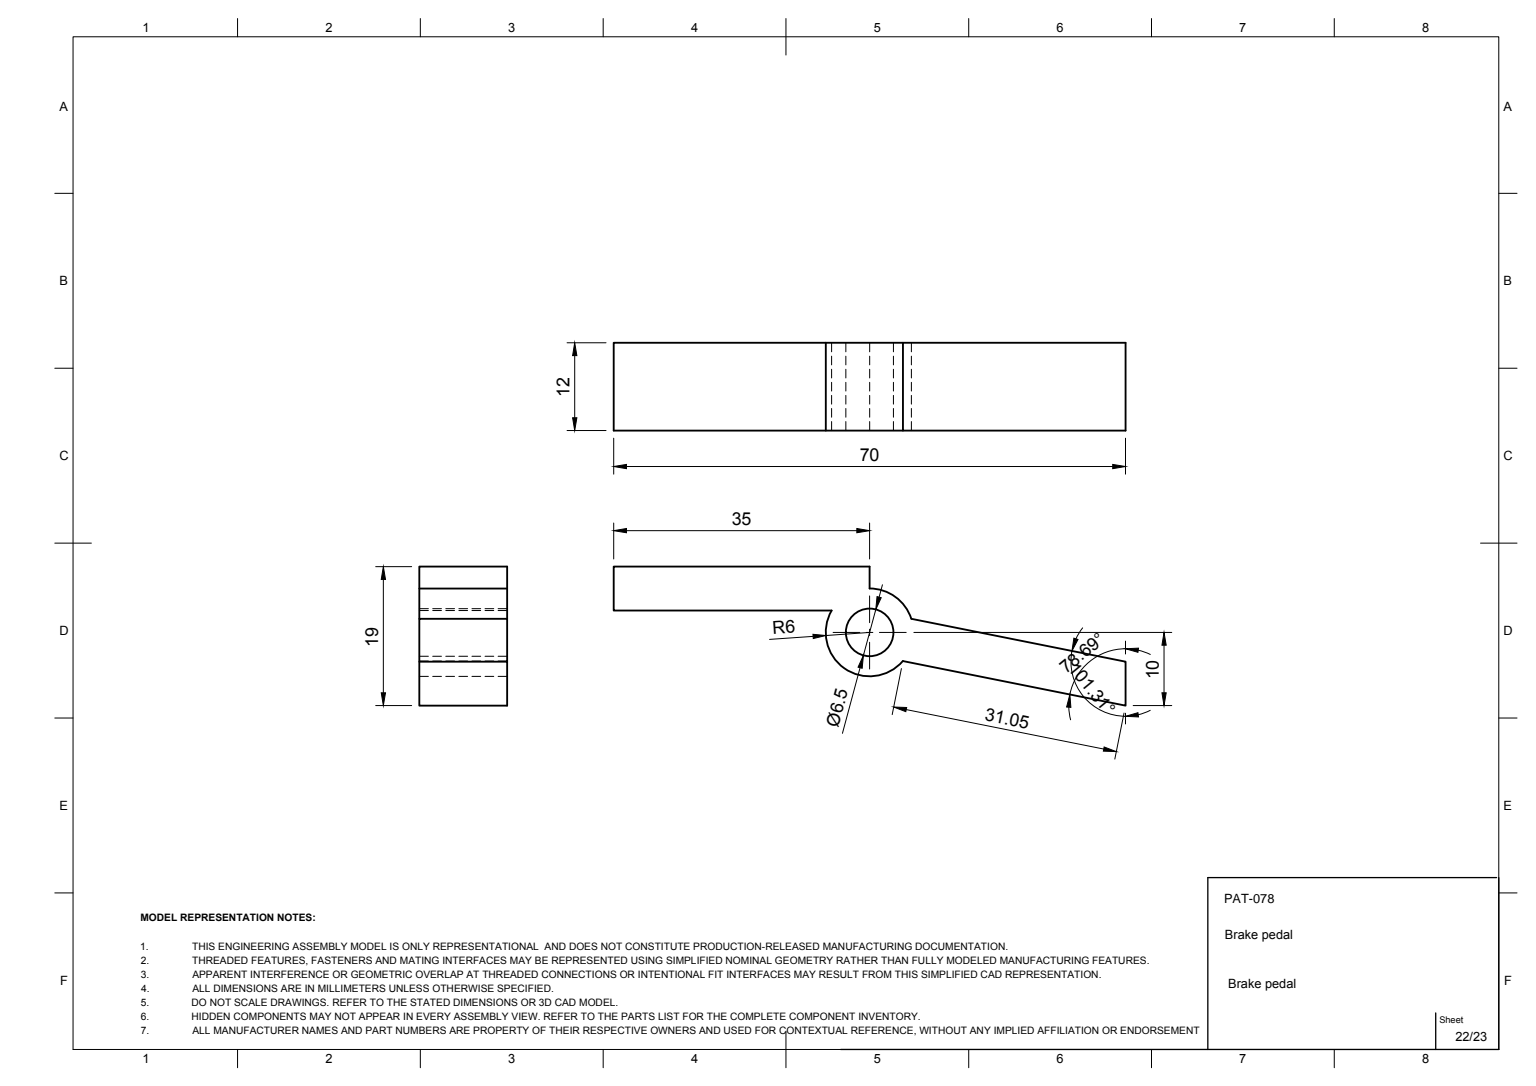
ISO-10303-21;
HEADER;
/* Generated by software containing ST-Developer
 * from STEP Tools, Inc. (www.steptools.com) 
 */

FILE_DESCRIPTION(
/* description */ ('Pedal-braked fixed caster'),
/* implementation_level */ '2;1');

FILE_NAME(
/* name */ 'Brake pedal.step',
/* time_stamp */ '2026-10-28T03:26:52-07:00',
/* author */ (''),
/* organization */ (''),
/* preprocessor_version */ 'ST-DEVELOPER v20.2',
/* originating_system */ 'Autodesk Translation Framework v15.17.0.0',
/* authorisation */ '');

FILE_SCHEMA (('AUTOMOTIVE_DESIGN { 1 0 10303 214 3 1 1 }'));
ENDSEC;

DATA;
#10=MECHANICAL_DESIGN_GEOMETRIC_PRESENTATION_REPRESENTATION('',(#228),#5734);
#187=SHAPE_REPRESENTATION_RELATIONSHIP('SRR','None',#5828,#204);
#204=ADVANCED_BREP_SHAPE_REPRESENTATION('',(#251),#5732);
#228=STYLED_ITEM('',(#5977),#251);
#251=MANIFOLD_SOLID_BREP('Body1',#3010);
#292=CYLINDRICAL_SURFACE('',#3531,0.325);
#293=CYLINDRICAL_SURFACE('',#3540,0.6);
#294=CYLINDRICAL_SURFACE('',#3548,0.6);
#338=FACE_BOUND('',#862,.T.);
#339=FACE_BOUND('',#869,.T.);
#470=CIRCLE('',#3532,0.325);
#471=CIRCLE('',#3533,0.325);
#472=CIRCLE('',#3538,0.6);
#473=CIRCLE('',#3539,0.6);
#474=CIRCLE('',#3541,0.6);
#475=CIRCLE('',#3547,0.6);
#636=FACE_OUTER_BOUND('',#857,.T.);
#637=FACE_OUTER_BOUND('',#858,.T.);
#638=FACE_OUTER_BOUND('',#859,.T.);
#639=FACE_OUTER_BOUND('',#860,.T.);
#640=FACE_OUTER_BOUND('',#861,.T.);
#641=FACE_OUTER_BOUND('',#863,.T.);
#642=FACE_OUTER_BOUND('',#864,.T.);
#643=FACE_OUTER_BOUND('',#865,.T.);
#644=FACE_OUTER_BOUND('',#866,.T.);
#645=FACE_OUTER_BOUND('',#867,.T.);
#646=FACE_OUTER_BOUND('',#868,.T.);
#647=FACE_OUTER_BOUND('',#870,.T.);
#857=EDGE_LOOP('',(#2616,#2617,#2618,#2619));
#858=EDGE_LOOP('',(#2620,#2621,#2622,#2623));
#859=EDGE_LOOP('',(#2624,#2625,#2626,#2627));
#860=EDGE_LOOP('',(#2628,#2629,#2630,#2631));
#861=EDGE_LOOP('',(#2632,#2633,#2634,#2635,#2636,#2637,#2638,#2639,#2640));
#862=EDGE_LOOP('',(#2641));
#863=EDGE_LOOP('',(#2642,#2643,#2644,#2645));
#864=EDGE_LOOP('',(#2646,#2647,#2648,#2649));
#865=EDGE_LOOP('',(#2650,#2651,#2652,#2653));
#866=EDGE_LOOP('',(#2654,#2655,#2656,#2657));
#867=EDGE_LOOP('',(#2658,#2659,#2660,#2661));
#868=EDGE_LOOP('',(#2662,#2663,#2664,#2665,#2666,#2667,#2668,#2669,#2670));
#869=EDGE_LOOP('',(#2671));
#870=EDGE_LOOP('',(#2672,#2673,#2674,#2675));
#1053=LINE('',#5599,#1265);
#1054=LINE('',#5604,#1266);
#1055=LINE('',#5606,#1267);
#1056=LINE('',#5608,#1268);
#1057=LINE('',#5609,#1269);
#1058=LINE('',#5612,#1270);
#1059=LINE('',#5614,#1271);
#1060=LINE('',#5615,#1272);
#1061=LINE('',#5619,#1273);
#1062=LINE('',#5620,#1274);
#1063=LINE('',#5621,#1275);
#1064=LINE('',#5626,#1276);
#1065=LINE('',#5628,#1277);
#1066=LINE('',#5630,#1278);
#1067=LINE('',#5632,#1279);
#1068=LINE('',#5637,#1280);
#1069=LINE('',#5640,#1281);
#1070=LINE('',#5642,#1282);
#1071=LINE('',#5643,#1283);
#1072=LINE('',#5646,#1284);
#1073=LINE('',#5647,#1285);
#1074=LINE('',#5650,#1286);
#1075=LINE('',#5651,#1287);
#1076=LINE('',#5653,#1288);
#1265=VECTOR('',#4403,0.325);
#1266=VECTOR('',#4408,1.);
#1267=VECTOR('',#4409,1.);
#1268=VECTOR('',#4410,1.);
#1269=VECTOR('',#4411,1.);
#1270=VECTOR('',#4414,1.);
#1271=VECTOR('',#4415,1.);
#1272=VECTOR('',#4416,1.);
#1273=VECTOR('',#4419,1.);
#1274=VECTOR('',#4420,1.);
#1275=VECTOR('',#4421,1.);
#1276=VECTOR('',#4426,1.);
#1277=VECTOR('',#4427,1.);
#1278=VECTOR('',#4428,1.);
#1279=VECTOR('',#4429,1.);
#1280=VECTOR('',#4436,1.);
#1281=VECTOR('',#4439,1.);
#1282=VECTOR('',#4440,1.);
#1283=VECTOR('',#4441,1.);
#1284=VECTOR('',#4444,1.);
#1285=VECTOR('',#4445,1.);
#1286=VECTOR('',#4448,1.);
#1287=VECTOR('',#4449,1.);
#1288=VECTOR('',#4452,1.);
#1532=VERTEX_POINT('',#5596);
#1533=VERTEX_POINT('',#5598);
#1534=VERTEX_POINT('',#5602);
#1535=VERTEX_POINT('',#5603);
#1536=VERTEX_POINT('',#5605);
#1537=VERTEX_POINT('',#5607);
#1538=VERTEX_POINT('',#5611);
#1539=VERTEX_POINT('',#5613);
#1540=VERTEX_POINT('',#5617);
#1541=VERTEX_POINT('',#5618);
#1542=VERTEX_POINT('',#5623);
#1543=VERTEX_POINT('',#5625);
#1544=VERTEX_POINT('',#5627);
#1545=VERTEX_POINT('',#5629);
#1546=VERTEX_POINT('',#5631);
#1547=VERTEX_POINT('',#5635);
#1548=VERTEX_POINT('',#5639);
#1549=VERTEX_POINT('',#5641);
#1550=VERTEX_POINT('',#5645);
#1551=VERTEX_POINT('',#5649);
#1898=EDGE_CURVE('',#1532,#1532,#470,.T.);
#1899=EDGE_CURVE('',#1532,#1533,#1053,.T.);
#1900=EDGE_CURVE('',#1533,#1533,#471,.T.);
#1901=EDGE_CURVE('',#1534,#1535,#1054,.T.);
#1902=EDGE_CURVE('',#1536,#1534,#1055,.T.);
#1903=EDGE_CURVE('',#1537,#1536,#1056,.T.);
#1904=EDGE_CURVE('',#1535,#1537,#1057,.T.);
#1905=EDGE_CURVE('',#1537,#1538,#1058,.T.);
#1906=EDGE_CURVE('',#1539,#1536,#1059,.T.);
#1907=EDGE_CURVE('',#1538,#1539,#1060,.T.);
#1908=EDGE_CURVE('',#1540,#1541,#1061,.T.);
#1909=EDGE_CURVE('',#1538,#1540,#1062,.T.);
#1910=EDGE_CURVE('',#1541,#1539,#1063,.T.);
#1911=EDGE_CURVE('',#1542,#1540,#472,.T.);
#1912=EDGE_CURVE('',#1542,#1543,#1064,.T.);
#1913=EDGE_CURVE('',#1543,#1544,#1065,.T.);
#1914=EDGE_CURVE('',#1544,#1545,#1066,.T.);
#1915=EDGE_CURVE('',#1545,#1546,#1067,.T.);
#1916=EDGE_CURVE('',#1535,#1546,#473,.T.);
#1917=EDGE_CURVE('',#1547,#1541,#474,.T.);
#1918=EDGE_CURVE('',#1547,#1542,#1068,.T.);
#1919=EDGE_CURVE('',#1546,#1548,#1069,.T.);
#1920=EDGE_CURVE('',#1545,#1549,#1070,.T.);
#1921=EDGE_CURVE('',#1548,#1549,#1071,.T.);
#1922=EDGE_CURVE('',#1550,#1547,#1072,.T.);
#1923=EDGE_CURVE('',#1543,#1550,#1073,.T.);
#1924=EDGE_CURVE('',#1551,#1550,#1074,.T.);
#1925=EDGE_CURVE('',#1544,#1551,#1075,.T.);
#1926=EDGE_CURVE('',#1549,#1551,#1076,.T.);
#1927=EDGE_CURVE('',#1534,#1548,#475,.T.);
#2616=ORIENTED_EDGE('',*,*,#1898,.F.);
#2617=ORIENTED_EDGE('',*,*,#1899,.T.);
#2618=ORIENTED_EDGE('',*,*,#1900,.F.);
#2619=ORIENTED_EDGE('',*,*,#1899,.F.);
#2620=ORIENTED_EDGE('',*,*,#1901,.F.);
#2621=ORIENTED_EDGE('',*,*,#1902,.F.);
#2622=ORIENTED_EDGE('',*,*,#1903,.F.);
#2623=ORIENTED_EDGE('',*,*,#1904,.F.);
#2624=ORIENTED_EDGE('',*,*,#1905,.F.);
#2625=ORIENTED_EDGE('',*,*,#1903,.T.);
#2626=ORIENTED_EDGE('',*,*,#1906,.F.);
#2627=ORIENTED_EDGE('',*,*,#1907,.F.);
#2628=ORIENTED_EDGE('',*,*,#1908,.F.);
#2629=ORIENTED_EDGE('',*,*,#1909,.F.);
#2630=ORIENTED_EDGE('',*,*,#1907,.T.);
#2631=ORIENTED_EDGE('',*,*,#1910,.F.);
#2632=ORIENTED_EDGE('',*,*,#1911,.F.);
#2633=ORIENTED_EDGE('',*,*,#1912,.T.);
#2634=ORIENTED_EDGE('',*,*,#1913,.T.);
#2635=ORIENTED_EDGE('',*,*,#1914,.T.);
#2636=ORIENTED_EDGE('',*,*,#1915,.T.);
#2637=ORIENTED_EDGE('',*,*,#1916,.F.);
#2638=ORIENTED_EDGE('',*,*,#1904,.T.);
#2639=ORIENTED_EDGE('',*,*,#1905,.T.);
#2640=ORIENTED_EDGE('',*,*,#1909,.T.);
#2641=ORIENTED_EDGE('',*,*,#1898,.T.);
#2642=ORIENTED_EDGE('',*,*,#1908,.T.);
#2643=ORIENTED_EDGE('',*,*,#1917,.F.);
#2644=ORIENTED_EDGE('',*,*,#1918,.T.);
#2645=ORIENTED_EDGE('',*,*,#1911,.T.);
#2646=ORIENTED_EDGE('',*,*,#1919,.F.);
#2647=ORIENTED_EDGE('',*,*,#1915,.F.);
#2648=ORIENTED_EDGE('',*,*,#1920,.T.);
#2649=ORIENTED_EDGE('',*,*,#1921,.F.);
#2650=ORIENTED_EDGE('',*,*,#1918,.F.);
#2651=ORIENTED_EDGE('',*,*,#1922,.F.);
#2652=ORIENTED_EDGE('',*,*,#1923,.F.);
#2653=ORIENTED_EDGE('',*,*,#1912,.F.);
#2654=ORIENTED_EDGE('',*,*,#1913,.F.);
#2655=ORIENTED_EDGE('',*,*,#1923,.T.);
#2656=ORIENTED_EDGE('',*,*,#1924,.F.);
#2657=ORIENTED_EDGE('',*,*,#1925,.F.);
#2658=ORIENTED_EDGE('',*,*,#1914,.F.);
#2659=ORIENTED_EDGE('',*,*,#1925,.T.);
#2660=ORIENTED_EDGE('',*,*,#1926,.F.);
#2661=ORIENTED_EDGE('',*,*,#1920,.F.);
#2662=ORIENTED_EDGE('',*,*,#1927,.T.);
#2663=ORIENTED_EDGE('',*,*,#1921,.T.);
#2664=ORIENTED_EDGE('',*,*,#1926,.T.);
#2665=ORIENTED_EDGE('',*,*,#1924,.T.);
#2666=ORIENTED_EDGE('',*,*,#1922,.T.);
#2667=ORIENTED_EDGE('',*,*,#1917,.T.);
#2668=ORIENTED_EDGE('',*,*,#1910,.T.);
#2669=ORIENTED_EDGE('',*,*,#1906,.T.);
#2670=ORIENTED_EDGE('',*,*,#1902,.T.);
#2671=ORIENTED_EDGE('',*,*,#1900,.T.);
#2672=ORIENTED_EDGE('',*,*,#1901,.T.);
#2673=ORIENTED_EDGE('',*,*,#1916,.T.);
#2674=ORIENTED_EDGE('',*,*,#1919,.T.);
#2675=ORIENTED_EDGE('',*,*,#1927,.F.);
#2794=PLANE('',#3534);
#2795=PLANE('',#3535);
#2796=PLANE('',#3536);
#2797=PLANE('',#3537);
#2798=PLANE('',#3542);
#2799=PLANE('',#3543);
#2800=PLANE('',#3544);
#2801=PLANE('',#3545);
#2802=PLANE('',#3546);
#2969=ADVANCED_FACE('',(#636),#292,.F.);
#2970=ADVANCED_FACE('',(#637),#2794,.T.);
#2971=ADVANCED_FACE('',(#638),#2795,.T.);
#2972=ADVANCED_FACE('',(#639),#2796,.T.);
#2973=ADVANCED_FACE('',(#640,#338),#2797,.F.);
#2974=ADVANCED_FACE('',(#641),#293,.T.);
#2975=ADVANCED_FACE('',(#642),#2798,.T.);
#2976=ADVANCED_FACE('',(#643),#2799,.T.);
#2977=ADVANCED_FACE('',(#644),#2800,.T.);
#2978=ADVANCED_FACE('',(#645),#2801,.T.);
#2979=ADVANCED_FACE('',(#646,#339),#2802,.T.);
#2980=ADVANCED_FACE('',(#647),#294,.T.);
#3010=CLOSED_SHELL('',(#2969,#2970,#2971,#2972,#2973,#2974,#2975,#2976,
#2977,#2978,#2979,#2980));
#3530=AXIS2_PLACEMENT_3D('',#5594,#4397,#4398);
#3531=AXIS2_PLACEMENT_3D('',#5595,#4399,#4400);
#3532=AXIS2_PLACEMENT_3D('',#5597,#4401,#4402);
#3533=AXIS2_PLACEMENT_3D('',#5600,#4404,#4405);
#3534=AXIS2_PLACEMENT_3D('',#5601,#4406,#4407);
#3535=AXIS2_PLACEMENT_3D('',#5610,#4412,#4413);
#3536=AXIS2_PLACEMENT_3D('',#5616,#4417,#4418);
#3537=AXIS2_PLACEMENT_3D('',#5622,#4422,#4423);
#3538=AXIS2_PLACEMENT_3D('',#5624,#4424,#4425);
#3539=AXIS2_PLACEMENT_3D('',#5633,#4430,#4431);
#3540=AXIS2_PLACEMENT_3D('',#5634,#4432,#4433);
#3541=AXIS2_PLACEMENT_3D('',#5636,#4434,#4435);
#3542=AXIS2_PLACEMENT_3D('',#5638,#4437,#4438);
#3543=AXIS2_PLACEMENT_3D('',#5644,#4442,#4443);
#3544=AXIS2_PLACEMENT_3D('',#5648,#4446,#4447);
#3545=AXIS2_PLACEMENT_3D('',#5652,#4450,#4451);
#3546=AXIS2_PLACEMENT_3D('',#5654,#4453,#4454);
#3547=AXIS2_PLACEMENT_3D('',#5655,#4455,#4456);
#3548=AXIS2_PLACEMENT_3D('',#5656,#4457,#4458);
#4397=DIRECTION('axis',(0.,0.,1.));
#4398=DIRECTION('refdir',(1.,0.,0.));
#4399=DIRECTION('center_axis',(0.,1.,0.));
#4400=DIRECTION('ref_axis',(1.,0.,0.));
#4401=DIRECTION('center_axis',(0.,1.,0.));
#4402=DIRECTION('ref_axis',(1.,0.,0.));
#4403=DIRECTION('',(0.,1.,0.));
#4404=DIRECTION('center_axis',(0.,-1.,0.));
#4405=DIRECTION('ref_axis',(1.,0.,0.));
#4406=DIRECTION('center_axis',(-0.196116135138184,0.,0.98058067569092));
#4407=DIRECTION('ref_axis',(0.98058067569092,0.,0.196116135138184));
#4408=DIRECTION('',(0.,-1.,0.));
#4409=DIRECTION('',(0.98058067569092,0.,0.196116135138184));
#4410=DIRECTION('',(0.,1.,0.));
#4411=DIRECTION('',(-0.98058067569092,0.,-0.196116135138184));
#4412=DIRECTION('center_axis',(-1.,0.,0.));
#4413=DIRECTION('ref_axis',(0.,0.,1.));
#4414=DIRECTION('',(0.,0.,-1.));
#4415=DIRECTION('',(0.,0.,1.));
#4416=DIRECTION('',(0.,1.,0.));
#4417=DIRECTION('center_axis',(0.196116135138184,0.,-0.98058067569092));
#4418=DIRECTION('ref_axis',(-0.98058067569092,0.,-0.196116135138184));
#4419=DIRECTION('',(0.,1.,0.));
#4420=DIRECTION('',(0.98058067569092,0.,0.196116135138184));
#4421=DIRECTION('',(-0.98058067569092,0.,-0.196116135138184));
#4422=DIRECTION('center_axis',(0.,1.,0.));
#4423=DIRECTION('ref_axis',(1.,0.,0.));
#4424=DIRECTION('center_axis',(0.,1.,0.));
#4425=DIRECTION('ref_axis',(1.,0.,0.));
#4426=DIRECTION('',(1.,0.,0.));
#4427=DIRECTION('',(0.,0.,1.));
#4428=DIRECTION('',(-1.,0.,0.));
#4429=DIRECTION('',(0.,0.,-1.));
#4430=DIRECTION('center_axis',(0.,1.,0.));
#4431=DIRECTION('ref_axis',(1.,0.,0.));
#4432=DIRECTION('center_axis',(0.,1.,0.));
#4433=DIRECTION('ref_axis',(1.,0.,0.));
#4434=DIRECTION('center_axis',(0.,1.,0.));
#4435=DIRECTION('ref_axis',(1.,0.,0.));
#4436=DIRECTION('',(0.,-1.,0.));
#4437=DIRECTION('center_axis',(-1.,0.,0.));
#4438=DIRECTION('ref_axis',(0.,0.,1.));
#4439=DIRECTION('',(0.,1.,0.));
#4440=DIRECTION('',(0.,1.,0.));
#4441=DIRECTION('',(0.,0.,1.));
#4442=DIRECTION('center_axis',(0.,0.,-1.));
#4443=DIRECTION('ref_axis',(-1.,0.,0.));
#4444=DIRECTION('',(-1.,0.,0.));
#4445=DIRECTION('',(0.,1.,0.));
#4446=DIRECTION('center_axis',(1.,0.,0.));
#4447=DIRECTION('ref_axis',(0.,0.,-1.));
#4448=DIRECTION('',(0.,0.,-1.));
#4449=DIRECTION('',(0.,1.,0.));
#4450=DIRECTION('center_axis',(0.,0.,1.));
#4451=DIRECTION('ref_axis',(1.,0.,0.));
#4452=DIRECTION('',(1.,0.,0.));
#4453=DIRECTION('center_axis',(0.,1.,0.));
#4454=DIRECTION('ref_axis',(1.,0.,0.));
#4455=DIRECTION('center_axis',(0.,1.,0.));
#4456=DIRECTION('ref_axis',(1.,0.,0.));
#4457=DIRECTION('center_axis',(0.,1.,0.));
#4458=DIRECTION('ref_axis',(1.,0.,0.));
#5594=CARTESIAN_POINT('',(0.,0.,0.));
#5595=CARTESIAN_POINT('Origin',(-3.,-0.7,9.));
#5596=CARTESIAN_POINT('',(-3.325,-0.6,9.));
#5597=CARTESIAN_POINT('Origin',(-3.,-0.6,9.));
#5598=CARTESIAN_POINT('',(-3.325,0.6,9.));
#5599=CARTESIAN_POINT('',(-3.325,-0.7,9.));
#5600=CARTESIAN_POINT('Origin',(-3.,0.6,9.));
#5601=CARTESIAN_POINT('Origin',(-6.5,-0.6,8.6));
#5602=CARTESIAN_POINT('',(-3.57047275484513,0.6,9.18590544903097));
#5603=CARTESIAN_POINT('',(-3.57047275484513,-0.6,9.18590544903098));
#5604=CARTESIAN_POINT('',(-3.57047275484513,-0.6,9.18590544903097));
#5605=CARTESIAN_POINT('',(-6.5,0.6,8.6));
#5606=CARTESIAN_POINT('',(-3.,0.6,9.3));
#5607=CARTESIAN_POINT('',(-6.5,-0.6,8.6));
#5608=CARTESIAN_POINT('',(-6.5,-0.6,8.6));
#5609=CARTESIAN_POINT('',(-3.,-0.6,9.3));
#5610=CARTESIAN_POINT('Origin',(-6.5,-0.6,8.));
#5611=CARTESIAN_POINT('',(-6.5,-0.6,8.));
#5612=CARTESIAN_POINT('',(-6.5,-0.6,8.6));
#5613=CARTESIAN_POINT('',(-6.5,0.6,8.));
#5614=CARTESIAN_POINT('',(-6.5,0.6,8.6));
#5615=CARTESIAN_POINT('',(-6.5,-0.6,8.));
#5616=CARTESIAN_POINT('Origin',(-3.,-0.6,8.7));
#5617=CARTESIAN_POINT('',(-3.45508813946051,-0.6,8.6089823721079));
#5618=CARTESIAN_POINT('',(-3.45508813946051,0.6,8.6089823721079));
#5619=CARTESIAN_POINT('',(-3.45508813946051,-0.6,8.6089823721079));
#5620=CARTESIAN_POINT('',(-6.5,-0.6,8.));
#5621=CARTESIAN_POINT('',(-6.5,0.6,8.));
#5622=CARTESIAN_POINT('Origin',(-3.,-0.6,9.));
#5623=CARTESIAN_POINT('',(-2.48038475772934,-0.6,9.3));
#5624=CARTESIAN_POINT('Origin',(-3.,-0.6,9.));
#5625=CARTESIAN_POINT('',(0.5,-0.6,9.3));
#5626=CARTESIAN_POINT('',(-3.,-0.6,9.3));
#5627=CARTESIAN_POINT('',(0.5,-0.6,9.9));
#5628=CARTESIAN_POINT('',(0.5,-0.6,9.3));
#5629=CARTESIAN_POINT('',(-3.,-0.6,9.9));
#5630=CARTESIAN_POINT('',(0.5,-0.6,9.9));
#5631=CARTESIAN_POINT('',(-3.,-0.6,9.6));
#5632=CARTESIAN_POINT('',(-3.,-0.6,9.9));
#5633=CARTESIAN_POINT('Origin',(-3.,-0.6,9.));
#5634=CARTESIAN_POINT('Origin',(-3.,-0.6,9.));
#5635=CARTESIAN_POINT('',(-2.48038475772934,0.6,9.3));
#5636=CARTESIAN_POINT('Origin',(-3.,0.6,9.));
#5637=CARTESIAN_POINT('',(-2.48038475772934,-0.6,9.3));
#5638=CARTESIAN_POINT('Origin',(-3.,-0.6,9.3));
#5639=CARTESIAN_POINT('',(-3.,0.6,9.6));
#5640=CARTESIAN_POINT('',(-3.,-0.6,9.6));
#5641=CARTESIAN_POINT('',(-3.,0.6,9.9));
#5642=CARTESIAN_POINT('',(-3.,-0.6,9.9));
#5643=CARTESIAN_POINT('',(-3.,0.6,9.9));
#5644=CARTESIAN_POINT('Origin',(0.5,-0.6,9.3));
#5645=CARTESIAN_POINT('',(0.5,0.6,9.3));
#5646=CARTESIAN_POINT('',(-3.,0.6,9.3));
#5647=CARTESIAN_POINT('',(0.5,-0.6,9.3));
#5648=CARTESIAN_POINT('Origin',(0.5,-0.6,9.9));
#5649=CARTESIAN_POINT('',(0.5,0.6,9.9));
#5650=CARTESIAN_POINT('',(0.5,0.6,9.3));
#5651=CARTESIAN_POINT('',(0.5,-0.6,9.9));
#5652=CARTESIAN_POINT('Origin',(-3.,-0.6,9.9));
#5653=CARTESIAN_POINT('',(0.5,0.6,9.9));
#5654=CARTESIAN_POINT('Origin',(-3.,0.6,9.));
#5655=CARTESIAN_POINT('Origin',(-3.,0.6,9.));
#5656=CARTESIAN_POINT('Origin',(-3.,-0.6,9.));
#5709=UNCERTAINTY_MEASURE_WITH_UNIT(LENGTH_MEASURE(0.001),#5735,
'DISTANCE_ACCURACY_VALUE',
'Maximum model space distance between geometric entities at asserted c
onnectivities');
#5711=UNCERTAINTY_MEASURE_WITH_UNIT(LENGTH_MEASURE(0.001),#5735,
'DISTANCE_ACCURACY_VALUE',
'Maximum model space distance between geometric entities at asserted c
onnectivities');
#5732=(
GEOMETRIC_REPRESENTATION_CONTEXT(3)
GLOBAL_UNCERTAINTY_ASSIGNED_CONTEXT((#5709))
GLOBAL_UNIT_ASSIGNED_CONTEXT((#5735,#5737,#5738))
REPRESENTATION_CONTEXT('','3D')
);
#5734=(
GEOMETRIC_REPRESENTATION_CONTEXT(3)
GLOBAL_UNCERTAINTY_ASSIGNED_CONTEXT((#5711))
GLOBAL_UNIT_ASSIGNED_CONTEXT((#5735,#5737,#5738))
REPRESENTATION_CONTEXT('','3D')
);
#5735=(
LENGTH_UNIT()
NAMED_UNIT(*)
SI_UNIT(.CENTI.,.METRE.)
);
#5737=(
NAMED_UNIT(*)
PLANE_ANGLE_UNIT()
SI_UNIT($,.RADIAN.)
);
#5738=(
NAMED_UNIT(*)
SI_UNIT($,.STERADIAN.)
SOLID_ANGLE_UNIT()
);
#5759=SHAPE_DEFINITION_REPRESENTATION(#5801,#5828);
#5801=PRODUCT_DEFINITION_SHAPE('',$,#5851);
#5828=SHAPE_REPRESENTATION('',(#3530),#5732);
#5830=PRODUCT_DEFINITION_CONTEXT('part definition',#5898,'design');
#5851=PRODUCT_DEFINITION('Brake pedal','Brake pedal',#5873,#5830);
#5873=PRODUCT_DEFINITION_FORMATION('',$,#5920);
#5898=APPLICATION_CONTEXT(
'Core Data for Automotive Mechanical Design Process');
#5899=PRODUCT_CONTEXT('part definition',#5898,'mechanical');
#5920=PRODUCT('Brake pedal','Brake pedal','Brake pedal',(#5899));
#5971=COLOUR_RGB('Sky Blue',0.24,0.69,0.87);
#5972=FILL_AREA_STYLE_COLOUR('',#5971);
#5973=FILL_AREA_STYLE('',(#5972));
#5974=SURFACE_STYLE_FILL_AREA(#5973);
#5975=SURFACE_SIDE_STYLE('',(#5974));
#5976=SURFACE_STYLE_USAGE(.BOTH.,#5975);
#5977=PRESENTATION_STYLE_ASSIGNMENT((#5976));
ENDSEC;
END-ISO-10303-21;
